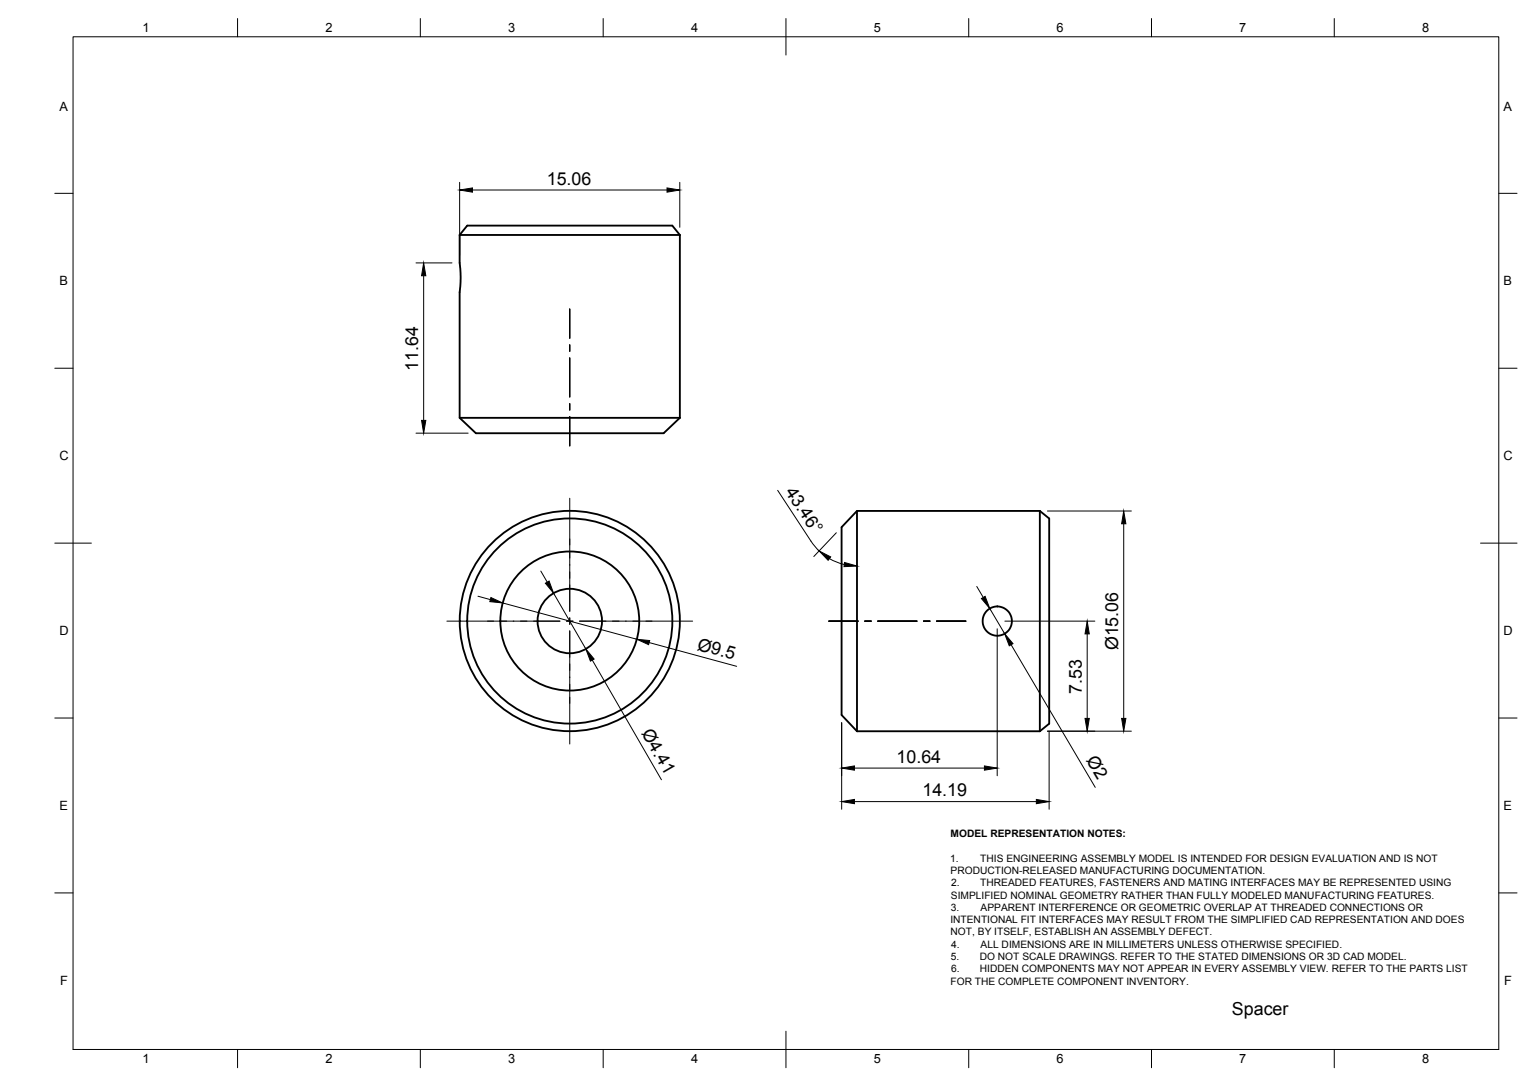
ISO-10303-21;
HEADER;
/* Generated by software containing ST-Developer
 * from STEP Tools, Inc. (www.steptools.com) 
 */

FILE_DESCRIPTION(
/* description */ (''),
/* implementation_level */ '2;1');

FILE_NAME(
/* name */ 'Spacer.step',
/* time_stamp */ '2026-10-06T13:15:55-07:00',
/* author */ (''),
/* organization */ (''),
/* preprocessor_version */ 'ST-DEVELOPER v20.2',
/* originating_system */ 'Autodesk Translation Framework v15.15.0.0',
/* authorisation */ '');

FILE_SCHEMA (('AUTOMOTIVE_DESIGN { 1 0 10303 214 3 1 1 }'));
ENDSEC;

DATA;
#10=MECHANICAL_DESIGN_GEOMETRIC_PRESENTATION_REPRESENTATION('',(#109),#27707);
#70=CONICAL_SURFACE('',#3978,7.269,0.680431320864525);
#71=CONICAL_SURFACE('',#3982,6.974,0.81226843236958);
#89=SHAPE_REPRESENTATION_RELATIONSHIP('SRR','None',#27746,#99);
#99=ADVANCED_BREP_SHAPE_REPRESENTATION('',(#119),#27698);
#109=STYLED_ITEM('',(#27804),#119);
#119=MANIFOLD_SOLID_BREP('Body1',#3835);
#130=FACE_BOUND('',#675,.T.);
#131=FACE_BOUND('',#677,.T.);
#132=FACE_BOUND('',#680,.T.);
#133=FACE_BOUND('',#683,.T.);
#134=FACE_BOUND('',#686,.T.);
#135=FACE_BOUND('',#689,.T.);
#171=PLANE('',#3976);
#172=PLANE('',#3984);
#173=PLANE('',#3988);
#174=PLANE('',#3992);
#222=CIRCLE('',#3974,4.75);
#223=CIRCLE('',#3975,4.75);
#224=CIRCLE('',#3977,7.01);
#225=CIRCLE('',#3979,7.528);
#226=CIRCLE('',#3981,7.528);
#227=CIRCLE('',#3983,6.42);
#228=CIRCLE('',#3985,3.7);
#229=CIRCLE('',#3987,3.7);
#230=CIRCLE('',#3989,2.204);
#231=CIRCLE('',#3991,2.204);
#346=CYLINDRICAL_SURFACE('',#3972,0.999999999999996);
#347=CYLINDRICAL_SURFACE('',#3973,4.75);
#348=CYLINDRICAL_SURFACE('',#3980,7.528);
#349=CYLINDRICAL_SURFACE('',#3986,3.7);
#350=CYLINDRICAL_SURFACE('',#3990,2.204);
#450=FACE_OUTER_BOUND('',#673,.T.);
#451=FACE_OUTER_BOUND('',#674,.T.);
#452=FACE_OUTER_BOUND('',#676,.T.);
#453=FACE_OUTER_BOUND('',#678,.T.);
#454=FACE_OUTER_BOUND('',#679,.T.);
#455=FACE_OUTER_BOUND('',#681,.T.);
#456=FACE_OUTER_BOUND('',#682,.T.);
#457=FACE_OUTER_BOUND('',#684,.T.);
#458=FACE_OUTER_BOUND('',#685,.T.);
#459=FACE_OUTER_BOUND('',#687,.T.);
#460=FACE_OUTER_BOUND('',#688,.T.);
#673=EDGE_LOOP('',(#2517,#2518,#2519,#2520,#2521,#2522));
#674=EDGE_LOOP('',(#2523,#2524,#2525,#2526));
#675=EDGE_LOOP('',(#2527,#2528));
#676=EDGE_LOOP('',(#2529));
#677=EDGE_LOOP('',(#2530));
#678=EDGE_LOOP('',(#2531,#2532,#2533,#2534));
#679=EDGE_LOOP('',(#2535,#2536,#2537,#2538));
#680=EDGE_LOOP('',(#2539,#2540));
#681=EDGE_LOOP('',(#2541,#2542,#2543,#2544));
#682=EDGE_LOOP('',(#2545));
#683=EDGE_LOOP('',(#2546));
#684=EDGE_LOOP('',(#2547,#2548,#2549,#2550));
#685=EDGE_LOOP('',(#2551));
#686=EDGE_LOOP('',(#2552));
#687=EDGE_LOOP('',(#2553,#2554,#2555,#2556));
#688=EDGE_LOOP('',(#2557));
#689=EDGE_LOOP('',(#2558));
#937=LINE('',#5341,#1113);
#938=LINE('',#5383,#1114);
#939=LINE('',#5391,#1115);
#940=LINE('',#5395,#1116);
#941=LINE('',#5398,#1117);
#942=LINE('',#5406,#1118);
#943=LINE('',#5413,#1119);
#1113=VECTOR('',#4346,0.999999999999996);
#1114=VECTOR('',#4351,4.75);
#1115=VECTOR('',#4362,7.269);
#1116=VECTOR('',#4367,7.528);
#1117=VECTOR('',#4370,6.974);
#1118=VECTOR('',#4381,3.7);
#1119=VECTOR('',#4390,2.204);
#1271=B_SPLINE_CURVE_WITH_KNOTS('',3,(#5304,#5305,#5306,#5307,#5308,#5309,
#5310,#5311,#5312,#5313,#5314,#5315,#5316,#5317,#5318,#5319,#5320,#5321,
#5322,#5323,#5324,#5325,#5326,#5327,#5328,#5329),.UNSPECIFIED.,.F.,.F.,
(4,2,2,2,2,2,2,2,2,2,2,2,4),(-0.604649456116834,-0.566857559730589,-0.529065663344343,
-0.491276377715985,-0.453487092087626,-0.415697806459267,-0.377908520830908,
-0.340116624444663,-0.302324728058417,-0.264532831672172,-0.226740935285926,
-0.188951649657567,-0.151162364029209),.UNSPECIFIED.);
#1272=B_SPLINE_CURVE_WITH_KNOTS('',3,(#5330,#5331,#5332,#5333,#5334,#5335,
#5336,#5337,#5338,#5339),.UNSPECIFIED.,.F.,.F.,(4,2,2,2,4),(-0.151162364029209,
-0.11337307840085,-0.0755837927724912,-0.0377918963862456,0.),
 .UNSPECIFIED.);
#1273=B_SPLINE_CURVE_WITH_KNOTS('',3,(#5343,#5344,#5345,#5346,#5347,#5348,
#5349,#5350,#5351,#5352),.UNSPECIFIED.,.F.,.F.,(4,2,2,2,4),(0.,0.037716777501004,
0.075433555002008,0.113149929875281,0.150866304748554),.UNSPECIFIED.);
#1274=B_SPLINE_CURVE_WITH_KNOTS('',3,(#5353,#5354,#5355,#5356,#5357,#5358,
#5359,#5360,#5361,#5362,#5363,#5364,#5365,#5366,#5367,#5368,#5369,#5370,
#5371,#5372,#5373,#5374,#5375,#5376,#5377,#5378),.UNSPECIFIED.,.F.,.F.,
(4,2,2,2,2,2,2,2,2,2,2,2,4),(0.150866304748554,0.188582679621827,0.2262990544951,
0.264015831996104,0.301732609497108,0.339449386998112,0.377166164499116,
0.414882539372389,0.452598914245662,0.490315289118935,0.528031663992208,
0.565748441493212,0.603465218994216),.UNSPECIFIED.);
#1541=VERTEX_POINT('',#5302);
#1542=VERTEX_POINT('',#5303);
#1543=VERTEX_POINT('',#5340);
#1544=VERTEX_POINT('',#5342);
#1545=VERTEX_POINT('',#5380);
#1546=VERTEX_POINT('',#5382);
#1547=VERTEX_POINT('',#5386);
#1548=VERTEX_POINT('',#5389);
#1549=VERTEX_POINT('',#5393);
#1550=VERTEX_POINT('',#5397);
#1551=VERTEX_POINT('',#5401);
#1552=VERTEX_POINT('',#5404);
#1553=VERTEX_POINT('',#5408);
#1554=VERTEX_POINT('',#5411);
#1928=EDGE_CURVE('',#1541,#1542,#1271,.T.);
#1929=EDGE_CURVE('',#1542,#1541,#1272,.T.);
#1930=EDGE_CURVE('',#1542,#1543,#937,.T.);
#1931=EDGE_CURVE('',#1544,#1543,#1273,.T.);
#1932=EDGE_CURVE('',#1543,#1544,#1274,.T.);
#1933=EDGE_CURVE('',#1545,#1545,#222,.T.);
#1934=EDGE_CURVE('',#1545,#1546,#938,.T.);
#1935=EDGE_CURVE('',#1546,#1546,#223,.T.);
#1936=EDGE_CURVE('',#1547,#1547,#224,.T.);
#1937=EDGE_CURVE('',#1548,#1548,#225,.T.);
#1938=EDGE_CURVE('',#1548,#1547,#939,.T.);
#1939=EDGE_CURVE('',#1549,#1549,#226,.T.);
#1940=EDGE_CURVE('',#1549,#1548,#940,.T.);
#1941=EDGE_CURVE('',#1549,#1550,#941,.T.);
#1942=EDGE_CURVE('',#1550,#1550,#227,.T.);
#1943=EDGE_CURVE('',#1551,#1551,#228,.T.);
#1944=EDGE_CURVE('',#1552,#1552,#229,.T.);
#1945=EDGE_CURVE('',#1552,#1551,#942,.T.);
#1946=EDGE_CURVE('',#1553,#1553,#230,.T.);
#1947=EDGE_CURVE('',#1554,#1554,#231,.T.);
#1948=EDGE_CURVE('',#1554,#1553,#943,.T.);
#2517=ORIENTED_EDGE('',*,*,#1928,.F.);
#2518=ORIENTED_EDGE('',*,*,#1929,.F.);
#2519=ORIENTED_EDGE('',*,*,#1930,.T.);
#2520=ORIENTED_EDGE('',*,*,#1931,.F.);
#2521=ORIENTED_EDGE('',*,*,#1932,.F.);
#2522=ORIENTED_EDGE('',*,*,#1930,.F.);
#2523=ORIENTED_EDGE('',*,*,#1933,.F.);
#2524=ORIENTED_EDGE('',*,*,#1934,.T.);
#2525=ORIENTED_EDGE('',*,*,#1935,.T.);
#2526=ORIENTED_EDGE('',*,*,#1934,.F.);
#2527=ORIENTED_EDGE('',*,*,#1928,.T.);
#2528=ORIENTED_EDGE('',*,*,#1929,.T.);
#2529=ORIENTED_EDGE('',*,*,#1936,.F.);
#2530=ORIENTED_EDGE('',*,*,#1933,.T.);
#2531=ORIENTED_EDGE('',*,*,#1937,.F.);
#2532=ORIENTED_EDGE('',*,*,#1938,.T.);
#2533=ORIENTED_EDGE('',*,*,#1936,.T.);
#2534=ORIENTED_EDGE('',*,*,#1938,.F.);
#2535=ORIENTED_EDGE('',*,*,#1939,.F.);
#2536=ORIENTED_EDGE('',*,*,#1940,.T.);
#2537=ORIENTED_EDGE('',*,*,#1937,.T.);
#2538=ORIENTED_EDGE('',*,*,#1940,.F.);
#2539=ORIENTED_EDGE('',*,*,#1931,.T.);
#2540=ORIENTED_EDGE('',*,*,#1932,.T.);
#2541=ORIENTED_EDGE('',*,*,#1939,.T.);
#2542=ORIENTED_EDGE('',*,*,#1941,.T.);
#2543=ORIENTED_EDGE('',*,*,#1942,.F.);
#2544=ORIENTED_EDGE('',*,*,#1941,.F.);
#2545=ORIENTED_EDGE('',*,*,#1942,.T.);
#2546=ORIENTED_EDGE('',*,*,#1943,.F.);
#2547=ORIENTED_EDGE('',*,*,#1944,.F.);
#2548=ORIENTED_EDGE('',*,*,#1945,.T.);
#2549=ORIENTED_EDGE('',*,*,#1943,.T.);
#2550=ORIENTED_EDGE('',*,*,#1945,.F.);
#2551=ORIENTED_EDGE('',*,*,#1944,.T.);
#2552=ORIENTED_EDGE('',*,*,#1946,.F.);
#2553=ORIENTED_EDGE('',*,*,#1947,.F.);
#2554=ORIENTED_EDGE('',*,*,#1948,.T.);
#2555=ORIENTED_EDGE('',*,*,#1946,.T.);
#2556=ORIENTED_EDGE('',*,*,#1948,.F.);
#2557=ORIENTED_EDGE('',*,*,#1935,.F.);
#2558=ORIENTED_EDGE('',*,*,#1947,.T.);
#3625=ADVANCED_FACE('',(#450),#346,.F.);
#3626=ADVANCED_FACE('',(#451,#130),#347,.F.);
#3627=ADVANCED_FACE('',(#452,#131),#171,.T.);
#3628=ADVANCED_FACE('',(#453),#70,.T.);
#3629=ADVANCED_FACE('',(#454,#132),#348,.T.);
#3630=ADVANCED_FACE('',(#455),#71,.T.);
#3631=ADVANCED_FACE('',(#456,#133),#172,.T.);
#3632=ADVANCED_FACE('',(#457),#349,.F.);
#3633=ADVANCED_FACE('',(#458,#134),#173,.T.);
#3634=ADVANCED_FACE('',(#459),#350,.F.);
#3635=ADVANCED_FACE('',(#460,#135),#174,.T.);
#3835=CLOSED_SHELL('',(#3625,#3626,#3627,#3628,#3629,#3630,#3631,#3632,
#3633,#3634,#3635));
#3971=AXIS2_PLACEMENT_3D('',#5300,#4342,#4343);
#3972=AXIS2_PLACEMENT_3D('',#5301,#4344,#4345);
#3973=AXIS2_PLACEMENT_3D('',#5379,#4347,#4348);
#3974=AXIS2_PLACEMENT_3D('',#5381,#4349,#4350);
#3975=AXIS2_PLACEMENT_3D('',#5384,#4352,#4353);
#3976=AXIS2_PLACEMENT_3D('',#5385,#4354,#4355);
#3977=AXIS2_PLACEMENT_3D('',#5387,#4356,#4357);
#3978=AXIS2_PLACEMENT_3D('',#5388,#4358,#4359);
#3979=AXIS2_PLACEMENT_3D('',#5390,#4360,#4361);
#3980=AXIS2_PLACEMENT_3D('',#5392,#4363,#4364);
#3981=AXIS2_PLACEMENT_3D('',#5394,#4365,#4366);
#3982=AXIS2_PLACEMENT_3D('',#5396,#4368,#4369);
#3983=AXIS2_PLACEMENT_3D('',#5399,#4371,#4372);
#3984=AXIS2_PLACEMENT_3D('',#5400,#4373,#4374);
#3985=AXIS2_PLACEMENT_3D('',#5402,#4375,#4376);
#3986=AXIS2_PLACEMENT_3D('',#5403,#4377,#4378);
#3987=AXIS2_PLACEMENT_3D('',#5405,#4379,#4380);
#3988=AXIS2_PLACEMENT_3D('',#5407,#4382,#4383);
#3989=AXIS2_PLACEMENT_3D('',#5409,#4384,#4385);
#3990=AXIS2_PLACEMENT_3D('',#5410,#4386,#4387);
#3991=AXIS2_PLACEMENT_3D('',#5412,#4388,#4389);
#3992=AXIS2_PLACEMENT_3D('',#5414,#4391,#4392);
#4342=DIRECTION('axis',(0.,0.,1.));
#4343=DIRECTION('refdir',(1.,0.,0.));
#4344=DIRECTION('center_axis',(0.,1.,0.));
#4345=DIRECTION('ref_axis',(1.,0.,0.));
#4346=DIRECTION('',(0.,1.,0.));
#4347=DIRECTION('center_axis',(1.,0.,0.));
#4348=DIRECTION('ref_axis',(0.,1.,0.));
#4349=DIRECTION('center_axis',(1.,0.,0.));
#4350=DIRECTION('ref_axis',(0.,0.,-1.));
#4351=DIRECTION('',(1.,0.,0.));
#4352=DIRECTION('center_axis',(1.,0.,0.));
#4353=DIRECTION('ref_axis',(0.,0.,-1.));
#4354=DIRECTION('center_axis',(-1.,0.,0.));
#4355=DIRECTION('ref_axis',(0.,0.,1.));
#4356=DIRECTION('center_axis',(1.,0.,0.));
#4357=DIRECTION('ref_axis',(0.,0.,-1.));
#4358=DIRECTION('center_axis',(1.,0.,0.));
#4359=DIRECTION('ref_axis',(0.,1.,0.));
#4360=DIRECTION('center_axis',(1.,0.,0.));
#4361=DIRECTION('ref_axis',(0.,0.,-1.));
#4362=DIRECTION('',(-0.777301434879696,0.629128348855753,7.70460018679057E-17));
#4363=DIRECTION('center_axis',(1.,0.,0.));
#4364=DIRECTION('ref_axis',(0.,1.,0.));
#4365=DIRECTION('center_axis',(1.,0.,0.));
#4366=DIRECTION('ref_axis',(0.,0.,-1.));
#4367=DIRECTION('',(-1.,0.,0.));
#4368=DIRECTION('center_axis',(-1.,0.,0.));
#4369=DIRECTION('ref_axis',(0.,1.,0.));
#4370=DIRECTION('',(0.687853663884889,0.725849390080431,-8.88909132225059E-17));
#4371=DIRECTION('center_axis',(1.,0.,0.));
#4372=DIRECTION('ref_axis',(0.,0.,-1.));
#4373=DIRECTION('center_axis',(1.,0.,0.));
#4374=DIRECTION('ref_axis',(0.,0.,-1.));
#4375=DIRECTION('center_axis',(1.,0.,0.));
#4376=DIRECTION('ref_axis',(0.,0.,-1.));
#4377=DIRECTION('center_axis',(1.,0.,0.));
#4378=DIRECTION('ref_axis',(0.,1.,0.));
#4379=DIRECTION('center_axis',(1.,0.,0.));
#4380=DIRECTION('ref_axis',(0.,0.,-1.));
#4381=DIRECTION('',(1.,0.,0.));
#4382=DIRECTION('center_axis',(1.,0.,0.));
#4383=DIRECTION('ref_axis',(0.,0.,-1.));
#4384=DIRECTION('center_axis',(1.,0.,0.));
#4385=DIRECTION('ref_axis',(0.,0.,-1.));
#4386=DIRECTION('center_axis',(1.,0.,0.));
#4387=DIRECTION('ref_axis',(0.,1.,0.));
#4388=DIRECTION('center_axis',(1.,0.,0.));
#4389=DIRECTION('ref_axis',(0.,0.,-1.));
#4390=DIRECTION('',(1.,0.,0.));
#4391=DIRECTION('center_axis',(-1.,0.,0.));
#4392=DIRECTION('ref_axis',(0.,0.,1.));
#5300=CARTESIAN_POINT('',(0.,0.,0.));
#5301=CARTESIAN_POINT('Origin',(70.8,0.,0.));
#5302=CARTESIAN_POINT('',(70.8,4.64354390525168,0.999999999999997));
#5303=CARTESIAN_POINT('',(69.8,4.75,-1.64281711919618E-16));
#5304=CARTESIAN_POINT('Ctrl Pts',(70.8,4.64354390525168,0.999999999999997));
#5305=CARTESIAN_POINT('Ctrl Pts',(70.9259729879541,4.64354390525168,0.999999999999997));
#5306=CARTESIAN_POINT('Ctrl Pts',(71.0600756275793,4.64920215672275,0.974746883632144));
#5307=CARTESIAN_POINT('Ctrl Pts',(71.3063376808864,4.66945597411313,0.872578382964584));
#5308=CARTESIAN_POINT('Ctrl Pts',(71.4185308600728,4.68373916194669,0.79568270230026));
#5309=CARTESIAN_POINT('Ctrl Pts',(71.5956765832561,4.71040703090821,0.618536979117035));
#5310=CARTESIAN_POINT('Ctrl Pts',(71.672577053022,4.72455080089029,0.50634121101625));
#5311=CARTESIAN_POINT('Ctrl Pts',(71.774749031943,4.74448366225285,0.260070124891274));
#5312=CARTESIAN_POINT('Ctrl Pts',(71.8,4.75,0.125964285427863));
#5313=CARTESIAN_POINT('Ctrl Pts',(71.8,4.75,-0.125964285427863));
#5314=CARTESIAN_POINT('Ctrl Pts',(71.774749031943,4.74448366225285,-0.260070124891274));
#5315=CARTESIAN_POINT('Ctrl Pts',(71.672577053022,4.72455080089029,-0.50634121101625));
#5316=CARTESIAN_POINT('Ctrl Pts',(71.5956765832561,4.71040703090821,-0.618536979117036));
#5317=CARTESIAN_POINT('Ctrl Pts',(71.4185308600728,4.68373916194669,-0.79568270230026));
#5318=CARTESIAN_POINT('Ctrl Pts',(71.3063376808864,4.66945597411313,-0.872578382964578));
#5319=CARTESIAN_POINT('Ctrl Pts',(71.0600756275793,4.64920215672275,-0.97474688363214));
#5320=CARTESIAN_POINT('Ctrl Pts',(70.9259729879542,4.64354390525168,-0.999999999999996));
#5321=CARTESIAN_POINT('Ctrl Pts',(70.6740270120459,4.64354390525168,-0.999999999999996));
#5322=CARTESIAN_POINT('Ctrl Pts',(70.5399243724207,4.64920215672275,-0.974746883632144));
#5323=CARTESIAN_POINT('Ctrl Pts',(70.2936623191136,4.66945597411312,-0.872578382964589));
#5324=CARTESIAN_POINT('Ctrl Pts',(70.1814691399272,4.68373916194669,-0.79568270230026));
#5325=CARTESIAN_POINT('Ctrl Pts',(70.0043234167439,4.71040703090821,-0.618536979117036));
#5326=CARTESIAN_POINT('Ctrl Pts',(69.927422946978,4.72455080089029,-0.50634121101625));
#5327=CARTESIAN_POINT('Ctrl Pts',(69.825250968057,4.74448366225285,-0.260070124891274));
#5328=CARTESIAN_POINT('Ctrl Pts',(69.8,4.75,-0.125964285427863));
#5329=CARTESIAN_POINT('Ctrl Pts',(69.8,4.75,-4.5102810375397E-16));
#5330=CARTESIAN_POINT('Ctrl Pts',(69.8,4.75,-1.38777878078145E-16));
#5331=CARTESIAN_POINT('Ctrl Pts',(69.8,4.75,0.125964285427862));
#5332=CARTESIAN_POINT('Ctrl Pts',(69.825250968057,4.74448366225285,0.260070124891274));
#5333=CARTESIAN_POINT('Ctrl Pts',(69.927422946978,4.72455080089029,0.50634121101625));
#5334=CARTESIAN_POINT('Ctrl Pts',(70.0043234167439,4.71040703090821,0.618536979117035));
#5335=CARTESIAN_POINT('Ctrl Pts',(70.1814691399272,4.68373916194669,0.79568270230026));
#5336=CARTESIAN_POINT('Ctrl Pts',(70.2936623191136,4.66945597411313,0.872578382964584));
#5337=CARTESIAN_POINT('Ctrl Pts',(70.5399243724207,4.64920215672275,0.974746883632144));
#5338=CARTESIAN_POINT('Ctrl Pts',(70.6740270120459,4.64354390525168,0.999999999999997));
#5339=CARTESIAN_POINT('Ctrl Pts',(70.8,4.64354390525168,0.999999999999997));
#5340=CARTESIAN_POINT('',(69.8,7.528,1.22464679914735E-16));
#5341=CARTESIAN_POINT('',(69.8,0.,1.22464679914735E-16));
#5342=CARTESIAN_POINT('',(70.8,7.46128568009562,0.999999999999996));
#5343=CARTESIAN_POINT('Ctrl Pts',(70.8,7.46128568009562,0.999999999999996));
#5344=CARTESIAN_POINT('Ctrl Pts',(70.67427740833,7.46128568009562,0.999999999999996));
#5345=CARTESIAN_POINT('Ctrl Pts',(70.540277592139,7.46479131730875,0.974843846039383));
#5346=CARTESIAN_POINT('Ctrl Pts',(70.2939429842273,7.4774158197129,0.87274427752583));
#5347=CARTESIAN_POINT('Ctrl Pts',(70.1815953412657,7.48634826149692,0.795808903638806));
#5348=CARTESIAN_POINT('Ctrl Pts',(70.004192043259,7.50308579458968,0.618405605632101));
#5349=CARTESIAN_POINT('Ctrl Pts',(69.9272559270855,7.51198372319629,0.506057551996159));
#5350=CARTESIAN_POINT('Ctrl Pts',(69.8251558158403,7.5245291161451,0.259721549521743));
#5351=CARTESIAN_POINT('Ctrl Pts',(69.8,7.528,0.125721249577576));
#5352=CARTESIAN_POINT('Ctrl Pts',(69.8,7.528,-3.46944695195361E-16));
#5353=CARTESIAN_POINT('Ctrl Pts',(69.8,7.528,-6.93889390390723E-17));
#5354=CARTESIAN_POINT('Ctrl Pts',(69.8,7.528,-0.125721249577577));
#5355=CARTESIAN_POINT('Ctrl Pts',(69.8251558158403,7.5245291161451,-0.259721549521743));
#5356=CARTESIAN_POINT('Ctrl Pts',(69.9272559270855,7.51198372319629,-0.506057551996159));
#5357=CARTESIAN_POINT('Ctrl Pts',(70.004192043259,7.50308579458968,-0.618405605632101));
#5358=CARTESIAN_POINT('Ctrl Pts',(70.1815953412657,7.48634826149692,-0.795808903638806));
#5359=CARTESIAN_POINT('Ctrl Pts',(70.2939429842273,7.4774158197129,-0.87274427752583));
#5360=CARTESIAN_POINT('Ctrl Pts',(70.540277592139,7.46479131730875,-0.974843846039383));
#5361=CARTESIAN_POINT('Ctrl Pts',(70.67427740833,7.46128568009562,-0.999999999999996));
#5362=CARTESIAN_POINT('Ctrl Pts',(70.92572259167,7.46128568009562,-0.999999999999996));
#5363=CARTESIAN_POINT('Ctrl Pts',(71.059722407861,7.46479131730875,-0.974843846039383));
#5364=CARTESIAN_POINT('Ctrl Pts',(71.3060570157727,7.4774158197129,-0.87274427752583));
#5365=CARTESIAN_POINT('Ctrl Pts',(71.4184046587343,7.48634826149692,-0.795808903638806));
#5366=CARTESIAN_POINT('Ctrl Pts',(71.595807956741,7.50308579458968,-0.618405605632101));
#5367=CARTESIAN_POINT('Ctrl Pts',(71.6727440729145,7.51198372319629,-0.506057551996159));
#5368=CARTESIAN_POINT('Ctrl Pts',(71.7748441841597,7.5245291161451,-0.259721549521743));
#5369=CARTESIAN_POINT('Ctrl Pts',(71.8,7.528,-0.125721249577577));
#5370=CARTESIAN_POINT('Ctrl Pts',(71.8,7.528,0.125721249577577));
#5371=CARTESIAN_POINT('Ctrl Pts',(71.7748441841597,7.5245291161451,0.259721549521733));
#5372=CARTESIAN_POINT('Ctrl Pts',(71.6727440729145,7.51198372319629,0.50605755199615));
#5373=CARTESIAN_POINT('Ctrl Pts',(71.595807956741,7.50308579458968,0.618405605632101));
#5374=CARTESIAN_POINT('Ctrl Pts',(71.4184046587343,7.48634826149692,0.795808903638806));
#5375=CARTESIAN_POINT('Ctrl Pts',(71.3060570157727,7.4774158197129,0.87274427752583));
#5376=CARTESIAN_POINT('Ctrl Pts',(71.059722407861,7.46479131730875,0.974843846039383));
#5377=CARTESIAN_POINT('Ctrl Pts',(70.92572259167,7.46128568009562,0.999999999999996));
#5378=CARTESIAN_POINT('Ctrl Pts',(70.8,7.46128568009562,0.999999999999996));
#5379=CARTESIAN_POINT('Origin',(69.875,0.,0.));
#5380=CARTESIAN_POINT('',(67.25,-4.75,-5.81707229594993E-16));
#5381=CARTESIAN_POINT('Origin',(67.25,0.,0.));
#5382=CARTESIAN_POINT('',(72.5,-4.75,-5.81707229594993E-16));
#5383=CARTESIAN_POINT('',(69.875,-4.75,-5.81707229594993E-16));
#5384=CARTESIAN_POINT('Origin',(72.5,0.,0.));
#5385=CARTESIAN_POINT('Origin',(67.25,7.01,0.));
#5386=CARTESIAN_POINT('',(67.25,-7.01,-8.58477406202294E-16));
#5387=CARTESIAN_POINT('Origin',(67.25,0.,0.));
#5388=CARTESIAN_POINT('Origin',(67.57,0.,0.));
#5389=CARTESIAN_POINT('',(67.89,-7.528,-9.21914110398127E-16));
#5390=CARTESIAN_POINT('Origin',(67.89,0.,0.));
#5391=CARTESIAN_POINT('',(67.57,-7.269,-8.90195758300211E-16));
#5392=CARTESIAN_POINT('Origin',(74.14,0.,0.));
#5393=CARTESIAN_POINT('',(80.39,-7.528,-9.21914110398127E-16));
#5394=CARTESIAN_POINT('Origin',(80.39,0.,0.));
#5395=CARTESIAN_POINT('',(74.14,-7.528,-9.21914110398128E-16));
#5396=CARTESIAN_POINT('Origin',(80.915,0.,0.));
#5397=CARTESIAN_POINT('',(81.44,-6.42,-7.86223245052601E-16));
#5398=CARTESIAN_POINT('',(80.915,-6.974,8.54068677725364E-16));
#5399=CARTESIAN_POINT('Origin',(81.44,0.,0.));
#5400=CARTESIAN_POINT('Origin',(81.44,3.7,0.));
#5401=CARTESIAN_POINT('',(81.44,-3.7,-4.53119315684521E-16));
#5402=CARTESIAN_POINT('Origin',(81.44,0.,0.));
#5403=CARTESIAN_POINT('Origin',(80.44,0.,0.));
#5404=CARTESIAN_POINT('',(79.44,-3.7,-4.53119315684521E-16));
#5405=CARTESIAN_POINT('Origin',(79.44,0.,0.));
#5406=CARTESIAN_POINT('',(80.44,-3.7,-4.53119315684521E-16));
#5407=CARTESIAN_POINT('Origin',(79.44,2.204,0.));
#5408=CARTESIAN_POINT('',(79.44,-2.204,-2.69912154532077E-16));
#5409=CARTESIAN_POINT('Origin',(79.44,0.,0.));
#5410=CARTESIAN_POINT('Origin',(75.97,0.,0.));
#5411=CARTESIAN_POINT('',(72.5,-2.204,-2.69912154532077E-16));
#5412=CARTESIAN_POINT('Origin',(72.5,0.,0.));
#5413=CARTESIAN_POINT('',(75.97,-2.204,-2.69912154532077E-16));
#5414=CARTESIAN_POINT('Origin',(72.5,4.75,0.));
#27686=UNCERTAINTY_MEASURE_WITH_UNIT(LENGTH_MEASURE(0.01),#27708,
'DISTANCE_ACCURACY_VALUE',
'Maximum model space distance between geometric entities at asserted c
onnectivities');
#27695=UNCERTAINTY_MEASURE_WITH_UNIT(LENGTH_MEASURE(0.01),#27708,
'DISTANCE_ACCURACY_VALUE',
'Maximum model space distance between geometric entities at asserted c
onnectivities');
#27698=(
GEOMETRIC_REPRESENTATION_CONTEXT(3)
GLOBAL_UNCERTAINTY_ASSIGNED_CONTEXT((#27686))
GLOBAL_UNIT_ASSIGNED_CONTEXT((#27708,#27710,#27711))
REPRESENTATION_CONTEXT('','3D')
);
#27707=(
GEOMETRIC_REPRESENTATION_CONTEXT(3)
GLOBAL_UNCERTAINTY_ASSIGNED_CONTEXT((#27695))
GLOBAL_UNIT_ASSIGNED_CONTEXT((#27708,#27710,#27711))
REPRESENTATION_CONTEXT('','3D')
);
#27708=(
LENGTH_UNIT()
NAMED_UNIT(*)
SI_UNIT(.MILLI.,.METRE.)
);
#27710=(
NAMED_UNIT(*)
PLANE_ANGLE_UNIT()
SI_UNIT($,.RADIAN.)
);
#27711=(
NAMED_UNIT(*)
SI_UNIT($,.STERADIAN.)
SOLID_ANGLE_UNIT()
);
#27714=SHAPE_DEFINITION_REPRESENTATION(#27725,#27746);
#27725=PRODUCT_DEFINITION_SHAPE('',$,#27758);
#27746=SHAPE_REPRESENTATION('',(#3971),#27698);
#27755=PRODUCT_DEFINITION_CONTEXT('part definition',#27790,'design');
#27758=PRODUCT_DEFINITION('spacer','Spacer',#27769,#27755);
#27769=PRODUCT_DEFINITION_FORMATION('',$,#27794);
#27790=APPLICATION_CONTEXT(
'Core Data for Automotive Mechanical Design Process');
#27791=PRODUCT_CONTEXT('part definition',#27790,'mechanical');
#27794=PRODUCT('spacer','Spacer',$,(#27791));
#27804=PRESENTATION_STYLE_ASSIGNMENT((#27806));
#27806=SURFACE_STYLE_USAGE(.BOTH.,#27808);
#27808=SURFACE_SIDE_STYLE('',(#27810));
#27810=SURFACE_STYLE_FILL_AREA(#27812);
#27812=FILL_AREA_STYLE('Opaque(160,160,160)',(#27814));
#27814=FILL_AREA_STYLE_COLOUR('Opaque(160,160,160)',#27816);
#27816=COLOUR_RGB('Opaque(160,160,160)', 0.09019608, 0.27058824, 0.51372549);
ENDSEC;
END-ISO-10303-21;
